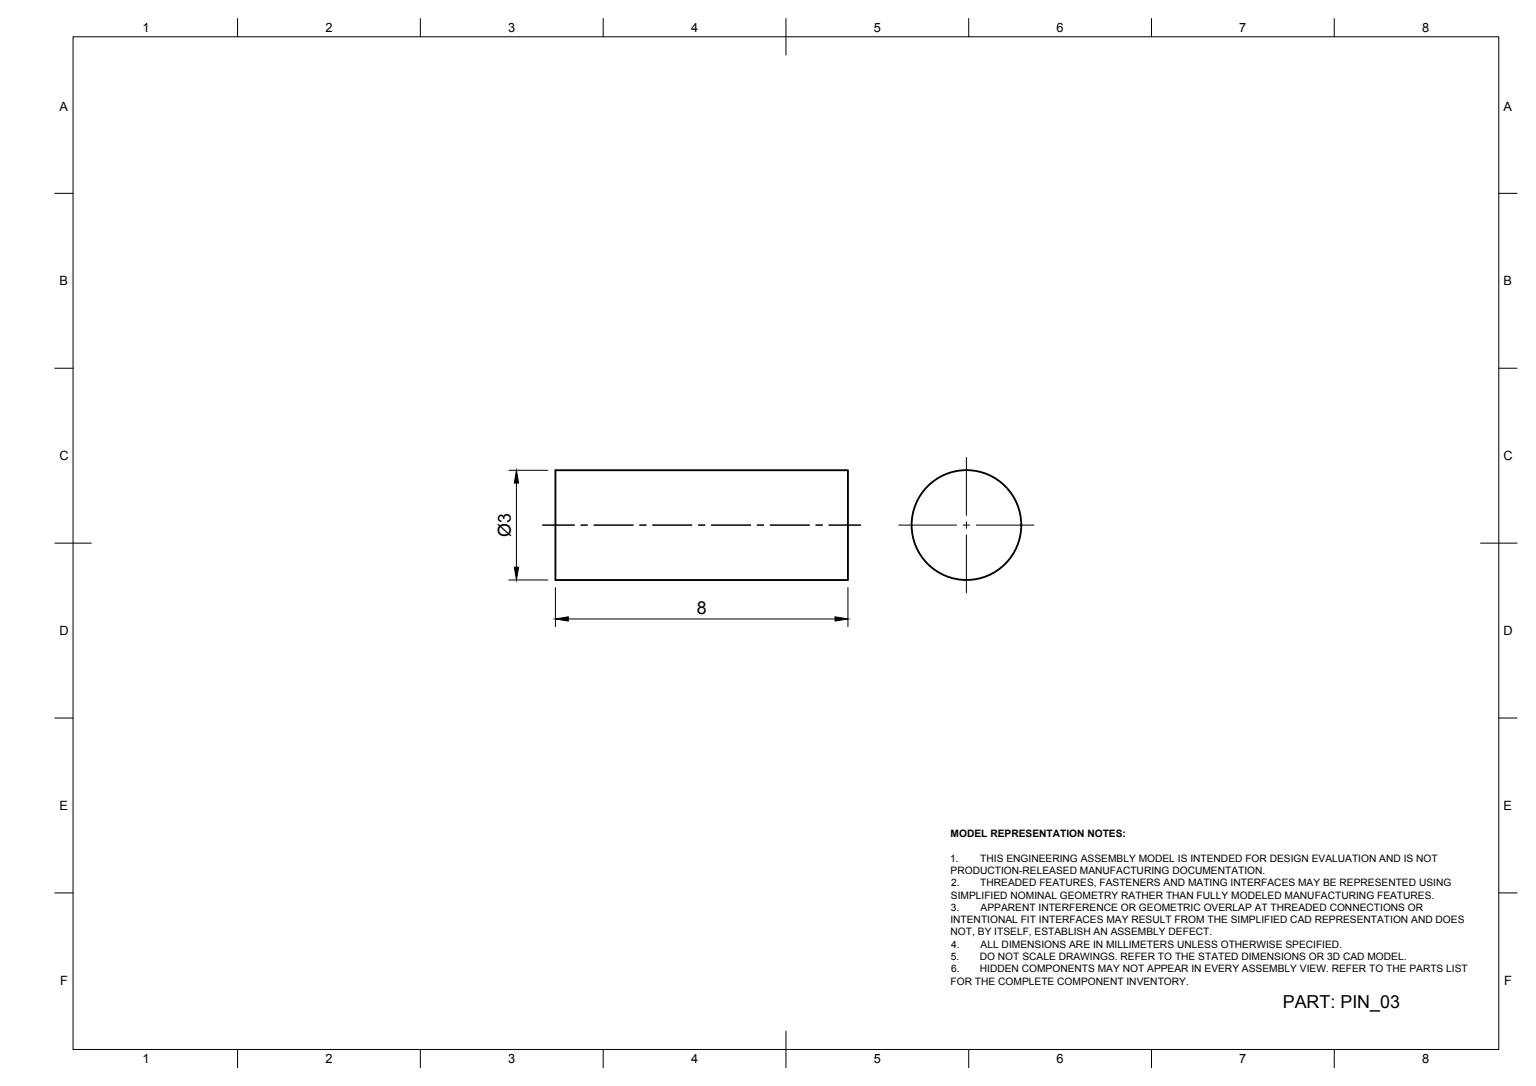
ISO-10303-21;
HEADER;
/* Generated by software containing ST-Developer
 * from STEP Tools, Inc. (www.steptools.com) 
 */

FILE_DESCRIPTION(
/* description */ (''),
/* implementation_level */ '2;1');

FILE_NAME(
/* name */ 'Pin_03.step',
/* time_stamp */ '2026-10-05T13:12:53-07:00',
/* author */ (''),
/* organization */ (''),
/* preprocessor_version */ 'ST-DEVELOPER v20.2',
/* originating_system */ 'Autodesk Translation Framework v15.15.0.0',
/* authorisation */ '');

FILE_SCHEMA (('AUTOMOTIVE_DESIGN { 1 0 10303 214 3 1 1 }'));
ENDSEC;

DATA;
#10=MECHANICAL_DESIGN_GEOMETRIC_PRESENTATION_REPRESENTATION('',(#62),#5912);
#46=SHAPE_REPRESENTATION_RELATIONSHIP('SRR','None',#5947,#54);
#54=ADVANCED_BREP_SHAPE_REPRESENTATION('',(#70),#5907);
#62=STYLED_ITEM('',(#5994),#70);
#70=MANIFOLD_SOLID_BREP('Body1',#3473);
#163=CYLINDRICAL_SURFACE('',#3849,1.4999996247669);
#335=FACE_OUTER_BOUND('',#538,.T.);
#336=FACE_OUTER_BOUND('',#539,.T.);
#337=FACE_OUTER_BOUND('',#540,.T.);
#538=EDGE_LOOP('',(#3130,#3131,#3132,#3133));
#539=EDGE_LOOP('',(#3134));
#540=EDGE_LOOP('',(#3135));
#645=CIRCLE('',#3850,1.4999996247669);
#646=CIRCLE('',#3851,1.4999996247669);
#1015=LINE('',#5845,#1380);
#1380=VECTOR('',#4814,1.4999996247669);
#1695=VERTEX_POINT('',#5842);
#1696=VERTEX_POINT('',#5844);
#2175=EDGE_CURVE('',#1695,#1695,#645,.T.);
#2176=EDGE_CURVE('',#1695,#1696,#1015,.T.);
#2177=EDGE_CURVE('',#1696,#1696,#646,.T.);
#3130=ORIENTED_EDGE('',*,*,#2175,.F.);
#3131=ORIENTED_EDGE('',*,*,#2176,.T.);
#3132=ORIENTED_EDGE('',*,*,#2177,.F.);
#3133=ORIENTED_EDGE('',*,*,#2176,.F.);
#3134=ORIENTED_EDGE('',*,*,#2177,.T.);
#3135=ORIENTED_EDGE('',*,*,#2175,.T.);
#3278=PLANE('',#3852);
#3279=PLANE('',#3853);
#3455=ADVANCED_FACE('',(#335),#163,.T.);
#3456=ADVANCED_FACE('',(#336),#3278,.T.);
#3457=ADVANCED_FACE('',(#337),#3279,.F.);
#3473=CLOSED_SHELL('',(#3455,#3456,#3457));
#3848=AXIS2_PLACEMENT_3D('',#5840,#4808,#4809);
#3849=AXIS2_PLACEMENT_3D('',#5841,#4810,#4811);
#3850=AXIS2_PLACEMENT_3D('',#5843,#4812,#4813);
#3851=AXIS2_PLACEMENT_3D('',#5846,#4815,#4816);
#3852=AXIS2_PLACEMENT_3D('',#5847,#4817,#4818);
#3853=AXIS2_PLACEMENT_3D('',#5848,#4819,#4820);
#4808=DIRECTION('axis',(0.,0.,1.));
#4809=DIRECTION('refdir',(1.,0.,0.));
#4810=DIRECTION('center_axis',(0.,-1.,0.));
#4811=DIRECTION('ref_axis',(-1.,0.,0.));
#4812=DIRECTION('center_axis',(1.83667601732677E-48,-1.,2.24927940568994E-64));
#4813=DIRECTION('ref_axis',(-1.,-1.83667601732677E-48,0.));
#4814=DIRECTION('',(0.,1.,0.));
#4815=DIRECTION('center_axis',(-1.83667601732677E-48,1.,-2.24927940568994E-64));
#4816=DIRECTION('ref_axis',(-1.,-1.83667601732677E-48,0.));
#4817=DIRECTION('center_axis',(-1.83667601732677E-48,1.,-2.24927940568994E-64));
#4818=DIRECTION('ref_axis',(-1.,-1.83667601732677E-48,0.));
#4819=DIRECTION('center_axis',(-1.83667601732677E-48,1.,-2.24927940568994E-64));
#4820=DIRECTION('ref_axis',(-1.,-1.83667601732677E-48,0.));
#5840=CARTESIAN_POINT('',(0.,0.,0.));
#5841=CARTESIAN_POINT('Origin',(100.979994297411,-4.00000000000001,103.500004749034));
#5842=CARTESIAN_POINT('',(102.479993922177,-12.,103.500004749034));
#5843=CARTESIAN_POINT('Origin',(100.979994297411,-12.,103.500004749034));
#5844=CARTESIAN_POINT('',(102.479993922177,-4.00000000000001,103.500004749034));
#5845=CARTESIAN_POINT('',(102.479993922178,-4.00000000000001,103.500004749034));
#5846=CARTESIAN_POINT('Origin',(100.979994297411,-4.00000000000001,103.500004749034));
#5847=CARTESIAN_POINT('Origin',(100.979994297411,-4.00000000000001,103.500004749034));
#5848=CARTESIAN_POINT('Origin',(100.979994297411,-12.,103.500004749034));
#5897=UNCERTAINTY_MEASURE_WITH_UNIT(LENGTH_MEASURE(0.01),#5913,
'DISTANCE_ACCURACY_VALUE',
'Maximum model space distance between geometric entities at asserted c
onnectivities');
#5902=UNCERTAINTY_MEASURE_WITH_UNIT(LENGTH_MEASURE(0.01),#5913,
'DISTANCE_ACCURACY_VALUE',
'Maximum model space distance between geometric entities at asserted c
onnectivities');
#5907=(
GEOMETRIC_REPRESENTATION_CONTEXT(3)
GLOBAL_UNCERTAINTY_ASSIGNED_CONTEXT((#5897))
GLOBAL_UNIT_ASSIGNED_CONTEXT((#5913,#5915,#5916))
REPRESENTATION_CONTEXT('','3D')
);
#5912=(
GEOMETRIC_REPRESENTATION_CONTEXT(3)
GLOBAL_UNCERTAINTY_ASSIGNED_CONTEXT((#5902))
GLOBAL_UNIT_ASSIGNED_CONTEXT((#5913,#5915,#5916))
REPRESENTATION_CONTEXT('','3D')
);
#5913=(
LENGTH_UNIT()
NAMED_UNIT(*)
SI_UNIT(.MILLI.,.METRE.)
);
#5915=(
NAMED_UNIT(*)
PLANE_ANGLE_UNIT()
SI_UNIT($,.RADIAN.)
);
#5916=(
NAMED_UNIT(*)
SI_UNIT($,.STERADIAN.)
SOLID_ANGLE_UNIT()
);
#5921=SHAPE_DEFINITION_REPRESENTATION(#5930,#5947);
#5930=PRODUCT_DEFINITION_SHAPE('',$,#5957);
#5947=SHAPE_REPRESENTATION('',(#3848),#5907);
#5952=PRODUCT_DEFINITION_CONTEXT('part definition',#5981,'design');
#5957=PRODUCT_DEFINITION('Pin_03','Pin_03',#5966,#5952);
#5966=PRODUCT_DEFINITION_FORMATION('',$,#5987);
#5981=APPLICATION_CONTEXT(
'Core Data for Automotive Mechanical Design Process');
#5982=PRODUCT_CONTEXT('part definition',#5981,'mechanical');
#5987=PRODUCT('Pin_03','Pin_03',$,(#5982));
#5994=PRESENTATION_STYLE_ASSIGNMENT((#5997));
#5997=SURFACE_STYLE_USAGE(.BOTH.,#6000);
#6000=SURFACE_SIDE_STYLE('',(#6003));
#6003=SURFACE_STYLE_FILL_AREA(#6006);
#6006=FILL_AREA_STYLE('Opaque(160,160,160)',(#6009));
#6009=FILL_AREA_STYLE_COLOUR('Opaque(160,160,160)',#6012);
#6012=COLOUR_RGB('Opaque(160,160,160)', 0.31764706, 0.68627451, 0.89019608);
ENDSEC;
END-ISO-10303-21;
